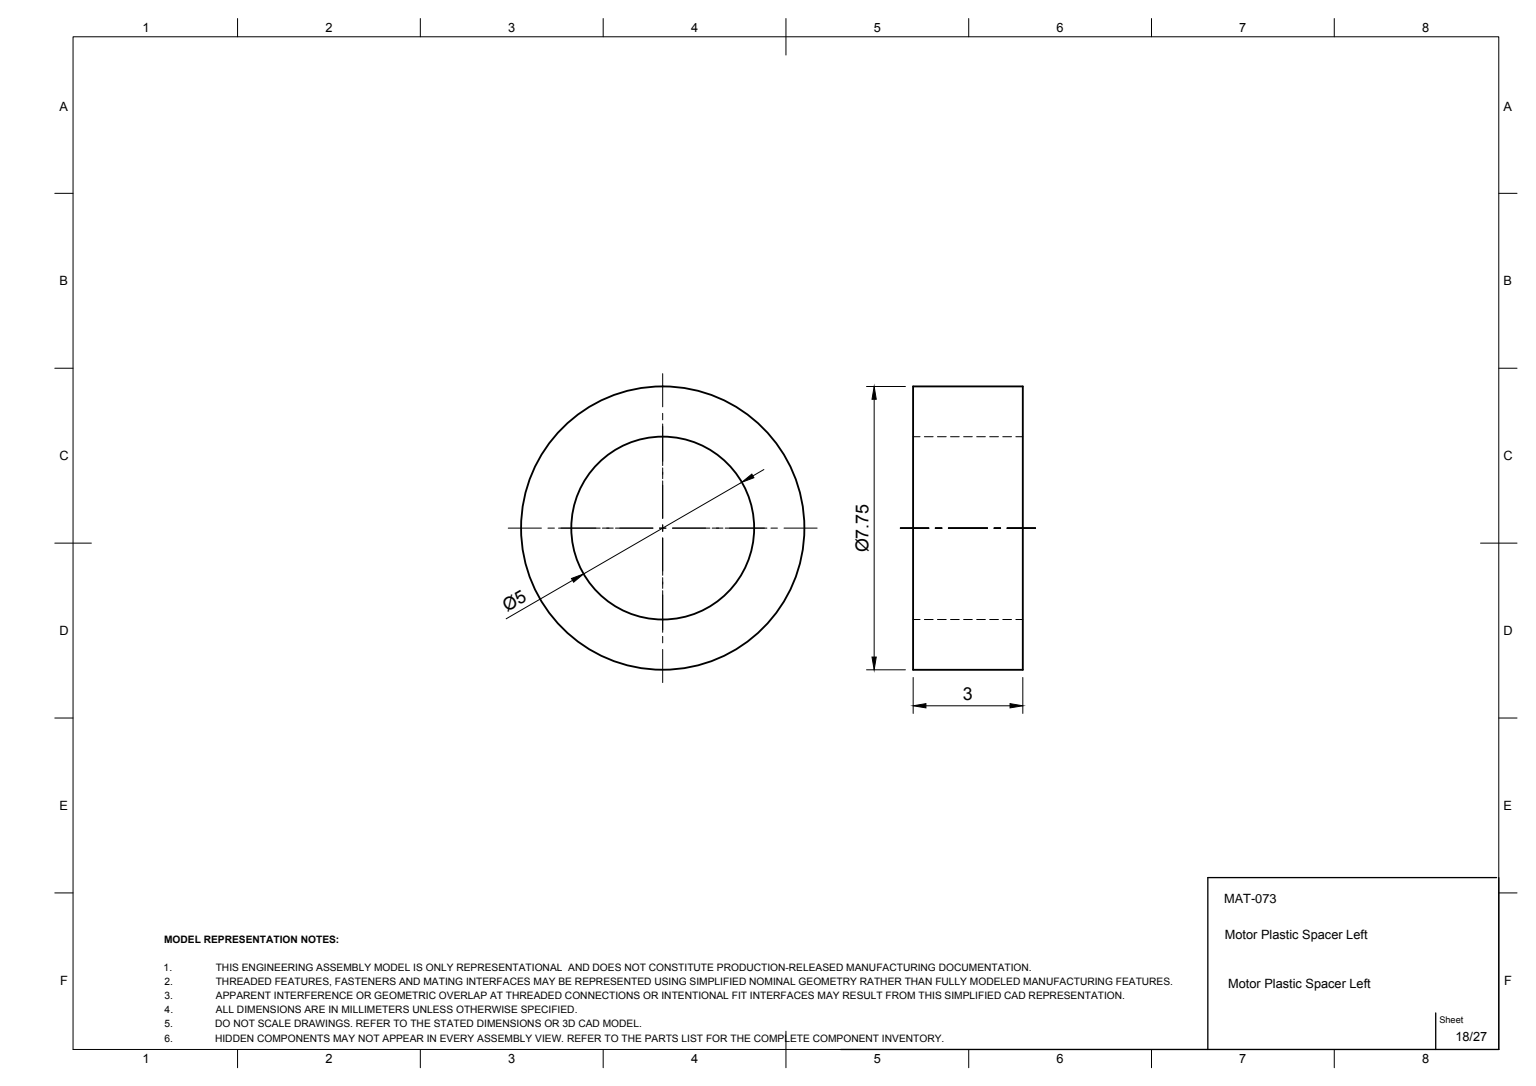
ISO-10303-21;
HEADER;
/* Generated by software containing ST-Developer
 * from STEP Tools, Inc. (www.steptools.com) 
 */

FILE_DESCRIPTION(
/* description */ ('CAx-IF Rec.Pracs.---Representation and Presentation of Product Manufa
cturing Information (PMI)---4.0---2014-10-13'),
/* implementation_level */ '2;1');

FILE_NAME(
/* name */ 'Motor Plastic Spacer Left.step',
/* time_stamp */ '2026-10-24T18:52:33-07:00',
/* author */ (''),
/* organization */ (''),
/* preprocessor_version */ 'ST-DEVELOPER v20.2',
/* originating_system */ 'Autodesk Translation Framework v15.17.0.0',
/* authorisation */ '');

FILE_SCHEMA (('AP242_MANAGED_MODEL_BASED_3D_ENGINEERING_MIM_LF { 1 0 10303 442 2 1 4 }'));
ENDSEC;

DATA;
#10=MECHANICAL_DESIGN_GEOMETRIC_PRESENTATION_REPRESENTATION('',(#432),#34876);
#366=SHAPE_REPRESENTATION_RELATIONSHIP('SRR','None',#35003,#399);
#399=ADVANCED_BREP_SHAPE_REPRESENTATION('',(#465),#34861);
#432=STYLED_ITEM('',(#35159),#465);
#465=MANIFOLD_SOLID_BREP('Motor Plastic Spacer Left',#19572);
#556=FACE_BOUND('',#6562,.T.);
#557=FACE_BOUND('',#6566,.T.);
#915=PLANE('',#21354);
#916=PLANE('',#21361);
#2062=LINE('',#32328,#3661);
#2063=LINE('',#32333,#3662);
#3661=VECTOR('',#26051,0.0025);
#3662=VECTOR('',#26058,0.003875);
#4585=CYLINDRICAL_SURFACE('',#21357,0.0025);
#4586=CYLINDRICAL_SURFACE('',#21359,0.003875);
#5440=FACE_OUTER_BOUND('',#6561,.T.);
#5441=FACE_OUTER_BOUND('',#6563,.T.);
#5442=FACE_OUTER_BOUND('',#6564,.T.);
#5443=FACE_OUTER_BOUND('',#6565,.T.);
#6561=EDGE_LOOP('',(#16280));
#6562=EDGE_LOOP('',(#16281));
#6563=EDGE_LOOP('',(#16282,#16283,#16284,#16285));
#6564=EDGE_LOOP('',(#16286,#16287,#16288,#16289));
#6565=EDGE_LOOP('',(#16290));
#6566=EDGE_LOOP('',(#16291));
#7617=CIRCLE('',#21355,0.00387500000001);
#7618=CIRCLE('',#21356,0.00250000000001);
#7619=CIRCLE('',#21358,0.00250000000001);
#7620=CIRCLE('',#21360,0.00387500000001);
#9223=VERTEX_POINT('',#32322);
#9224=VERTEX_POINT('',#32324);
#9225=VERTEX_POINT('',#32327);
#9226=VERTEX_POINT('',#32331);
#11698=EDGE_CURVE('',#9223,#9223,#7617,.T.);
#11699=EDGE_CURVE('',#9224,#9224,#7618,.T.);
#11700=EDGE_CURVE('',#9224,#9225,#2062,.T.);
#11701=EDGE_CURVE('',#9225,#9225,#7619,.T.);
#11702=EDGE_CURVE('',#9226,#9226,#7620,.T.);
#11703=EDGE_CURVE('',#9226,#9223,#2063,.T.);
#16280=ORIENTED_EDGE('',*,*,#11698,.T.);
#16281=ORIENTED_EDGE('',*,*,#11699,.T.);
#16282=ORIENTED_EDGE('',*,*,#11699,.F.);
#16283=ORIENTED_EDGE('',*,*,#11700,.T.);
#16284=ORIENTED_EDGE('',*,*,#11701,.F.);
#16285=ORIENTED_EDGE('',*,*,#11700,.F.);
#16286=ORIENTED_EDGE('',*,*,#11702,.F.);
#16287=ORIENTED_EDGE('',*,*,#11703,.T.);
#16288=ORIENTED_EDGE('',*,*,#11698,.F.);
#16289=ORIENTED_EDGE('',*,*,#11703,.F.);
#16290=ORIENTED_EDGE('',*,*,#11702,.T.);
#16291=ORIENTED_EDGE('',*,*,#11701,.T.);
#19156=ADVANCED_FACE('',(#5440,#556),#915,.F.);
#19157=ADVANCED_FACE('',(#5441),#4585,.F.);
#19158=ADVANCED_FACE('',(#5442),#4586,.T.);
#19159=ADVANCED_FACE('',(#5443,#557),#916,.T.);
#19572=CLOSED_SHELL('',(#19156,#19157,#19158,#19159));
#21353=AXIS2_PLACEMENT_3D('',#32320,#26041,#26042);
#21354=AXIS2_PLACEMENT_3D('',#32321,#26043,#26044);
#21355=AXIS2_PLACEMENT_3D('',#32323,#26045,#26046);
#21356=AXIS2_PLACEMENT_3D('',#32325,#26047,#26048);
#21357=AXIS2_PLACEMENT_3D('',#32326,#26049,#26050);
#21358=AXIS2_PLACEMENT_3D('',#32329,#26052,#26053);
#21359=AXIS2_PLACEMENT_3D('',#32330,#26054,#26055);
#21360=AXIS2_PLACEMENT_3D('',#32332,#26056,#26057);
#21361=AXIS2_PLACEMENT_3D('',#32334,#26059,#26060);
#26041=DIRECTION('axis',(0.,0.,1.));
#26042=DIRECTION('refdir',(1.,0.,0.));
#26043=DIRECTION('center_axis',(0.,1.,0.));
#26044=DIRECTION('ref_axis',(1.,0.,0.));
#26045=DIRECTION('center_axis',(0.,-1.,0.));
#26046=DIRECTION('ref_axis',(-1.,0.,0.));
#26047=DIRECTION('center_axis',(0.,1.,0.));
#26048=DIRECTION('ref_axis',(1.,0.,0.));
#26049=DIRECTION('center_axis',(0.,1.,0.));
#26050=DIRECTION('ref_axis',(1.,0.,0.));
#26051=DIRECTION('',(0.,1.,0.));
#26052=DIRECTION('center_axis',(0.,-1.,0.));
#26053=DIRECTION('ref_axis',(1.,0.,0.));
#26054=DIRECTION('center_axis',(0.,1.,0.));
#26055=DIRECTION('ref_axis',(-1.,0.,0.));
#26056=DIRECTION('center_axis',(0.,1.,0.));
#26057=DIRECTION('ref_axis',(-1.,0.,0.));
#26058=DIRECTION('',(0.,-1.,0.));
#26059=DIRECTION('center_axis',(0.,1.,0.));
#26060=DIRECTION('ref_axis',(1.,0.,0.));
#32320=CARTESIAN_POINT('',(0.,0.,0.));
#32321=CARTESIAN_POINT('Origin',(-4.59950432489715E-17,-0.01,1.1450674770076E-32));
#32322=CARTESIAN_POINT('',(0.00387499999999995,-0.01000000000001,-4.74550634669588E-19));
#32323=CARTESIAN_POINT('Origin',(-4.59950432489715E-17,-0.01000000000001,
1.1450674770076E-32));
#32324=CARTESIAN_POINT('',(-0.00250000000000005,-0.01000000000001,3.0616169978685E-19));
#32325=CARTESIAN_POINT('Origin',(-4.59950432489715E-17,-0.01000000000001,
1.1450674770076E-32));
#32326=CARTESIAN_POINT('Origin',(-4.59950432489715E-17,-0.0085,1.1450674770076E-32));
#32327=CARTESIAN_POINT('',(-0.00250000000000005,-0.00699999999999,3.0616169978685E-19));
#32328=CARTESIAN_POINT('',(-0.00250000000000005,-0.0085,3.0616169978685E-19));
#32329=CARTESIAN_POINT('Origin',(-4.59950432489715E-17,-0.00699999999999,
1.1450674770076E-32));
#32330=CARTESIAN_POINT('Origin',(-4.59950432489715E-17,-0.0085,1.1450674770076E-32));
#32331=CARTESIAN_POINT('',(0.00387499999999995,-0.00699999999999,-4.74550634669588E-19));
#32332=CARTESIAN_POINT('Origin',(-4.59950432489715E-17,-0.00699999999999,
1.1450674770076E-32));
#32333=CARTESIAN_POINT('',(0.00387499999999995,-0.0085,-4.74550634669588E-19));
#32334=CARTESIAN_POINT('Origin',(-4.59950432489715E-17,-0.007,1.1450674770076E-32));
#34826=UNCERTAINTY_MEASURE_WITH_UNIT(LENGTH_MEASURE(1.E-5),#34877,
'DISTANCE_ACCURACY_VALUE',
'Maximum model space distance between geometric entities at asserted c
onnectivities');
#34841=UNCERTAINTY_MEASURE_WITH_UNIT(LENGTH_MEASURE(1.E-5),#34877,
'DISTANCE_ACCURACY_VALUE',
'Maximum model space distance between geometric entities at asserted c
onnectivities');
#34861=(
GEOMETRIC_REPRESENTATION_CONTEXT(3)
GLOBAL_UNCERTAINTY_ASSIGNED_CONTEXT((#34826))
GLOBAL_UNIT_ASSIGNED_CONTEXT((#34877,#34878,#34879))
REPRESENTATION_CONTEXT('','3D')
);
#34876=(
GEOMETRIC_REPRESENTATION_CONTEXT(3)
GLOBAL_UNCERTAINTY_ASSIGNED_CONTEXT((#34841))
GLOBAL_UNIT_ASSIGNED_CONTEXT((#34877,#34878,#34879))
REPRESENTATION_CONTEXT('','3D')
);
#34877=(
LENGTH_UNIT()
NAMED_UNIT(*)
SI_UNIT($,.METRE.)
);
#34878=(
NAMED_UNIT(*)
PLANE_ANGLE_UNIT()
SI_UNIT($,.RADIAN.)
);
#34879=(
NAMED_UNIT(*)
SI_UNIT($,.STERADIAN.)
SOLID_ANGLE_UNIT()
);
#34899=SHAPE_DEFINITION_REPRESENTATION(#34933,#35003);
#34933=PRODUCT_DEFINITION_SHAPE('',$,#35038);
#35003=SHAPE_REPRESENTATION('',(#21353),#34861);
#35018=PRODUCT_DEFINITION_CONTEXT('part definition',#35122,'design');
#35038=PRODUCT_DEFINITION('Motor Plastic Spacer Left',
'Motor Plastic Spacer Left',#35072,#35018);
#35072=PRODUCT_DEFINITION_FORMATION('',$,#35143);
#35122=APPLICATION_CONTEXT('Managed model based 3d engineering');
#35123=PRODUCT_CONTEXT('part definition',#35122,'mechanical');
#35143=PRODUCT('Motor Plastic Spacer Left','Motor Plastic Spacer Left',

'LEGAL AND USAGE DISCLAIMER: this Data/Model is provided \X2\201C\X0\A
S IS\X2\201D\X0\ for informational and representational only. It is a 
geometric approximation and is NOT engineered, certified, or guarantee
d for dimensional accuracy, exact tolerances, or production-level prec
ision. Vendor disclaims all implied warranties including fitness for a
 particular purpose. DO NOT USE FOR DIRECT PHYSICAL MANUFACTURING, AUT
OMATED PRODUCTION, OR SAFETY-CRITICAL SYSTEMS without independent engi
neering verification and resolution of any design discrepancies.',(#35123));
#35159=PRESENTATION_STYLE_ASSIGNMENT((#35168));
#35168=SURFACE_STYLE_USAGE(.BOTH.,#35177);
#35177=SURFACE_SIDE_STYLE('',(#35186));
#35186=SURFACE_STYLE_FILL_AREA(#35195);
#35195=FILL_AREA_STYLE('Paint - Enamel Glossy (White)',(#35204));
#35204=FILL_AREA_STYLE_COLOUR('Paint - Enamel Glossy (White)',#35213);
#35213=COLOUR_RGB('Paint - Enamel Glossy (White)',0.964705882352941,0.964705882352941,
0.952941176470588);
ENDSEC;
END-ISO-10303-21;
